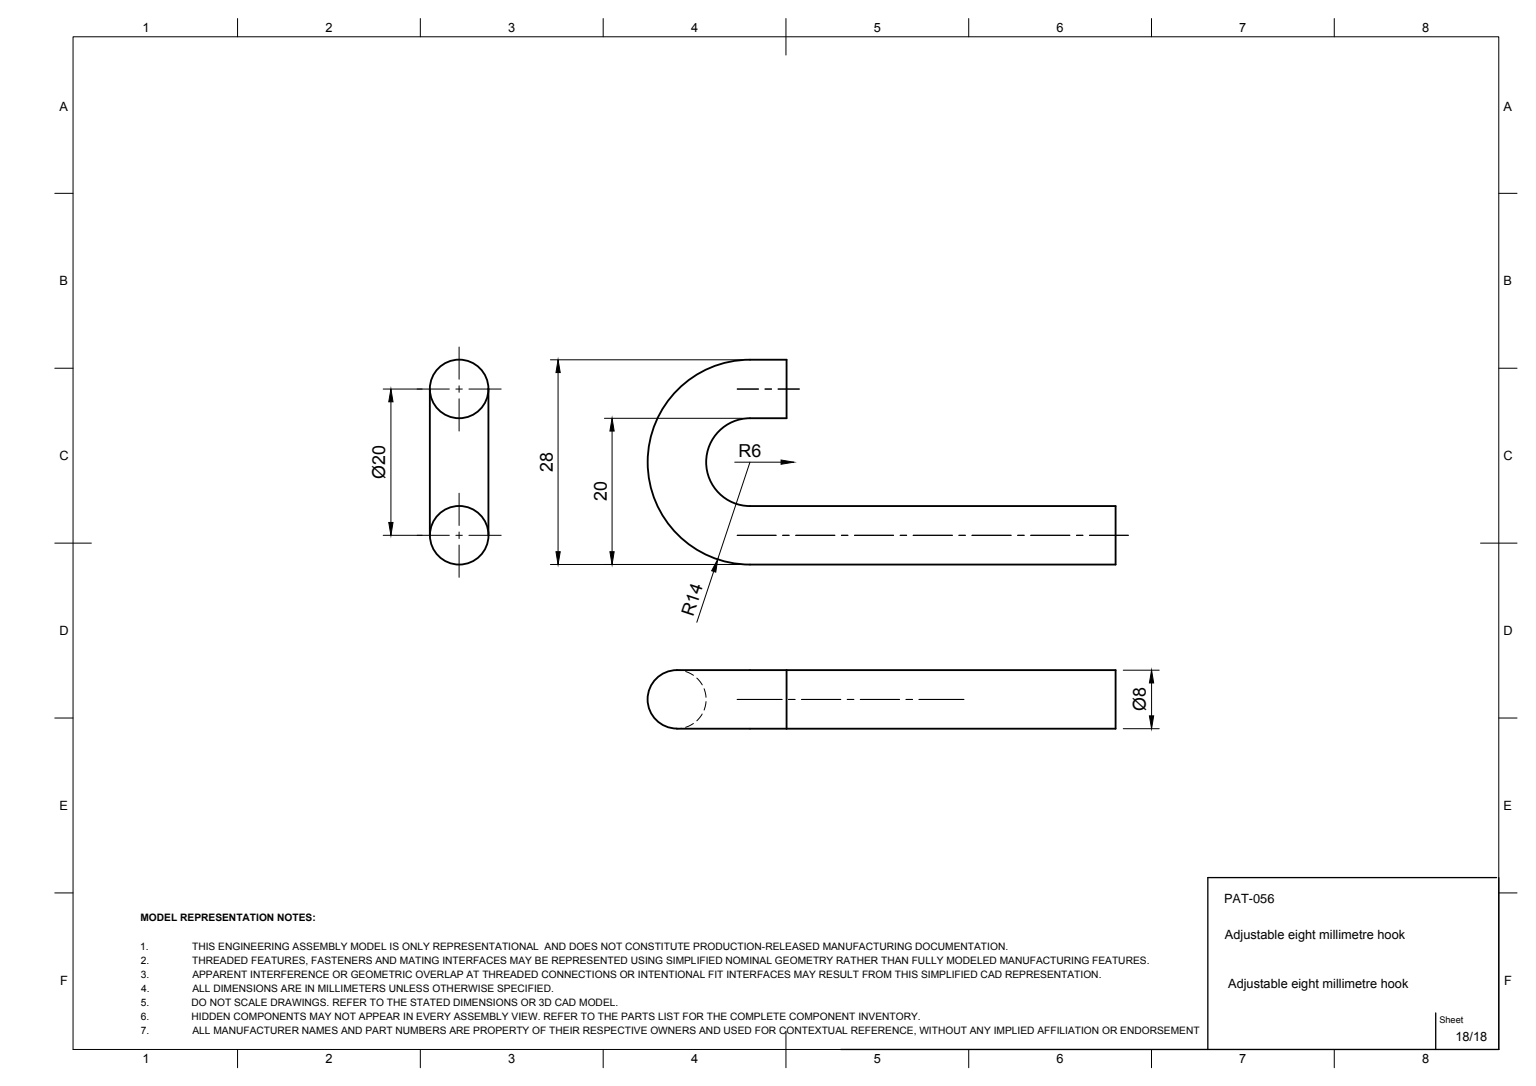
ISO-10303-21;
HEADER;
/* Generated by software containing ST-Developer
 * from STEP Tools, Inc. (www.steptools.com) 
 */

FILE_DESCRIPTION(
/* description */ ('Hook toggle clamp'),
/* implementation_level */ '2;1');

FILE_NAME(
/* name */ 'Adjustable eight millimetre hook.step',
/* time_stamp */ '2026-10-27T21:56:56-07:00',
/* author */ (''),
/* organization */ (''),
/* preprocessor_version */ 'ST-DEVELOPER v20.2',
/* originating_system */ 'Autodesk Translation Framework v15.17.0.0',
/* authorisation */ '');

FILE_SCHEMA (('AUTOMOTIVE_DESIGN { 1 0 10303 214 3 1 1 }'));
ENDSEC;

DATA;
#10=MECHANICAL_DESIGN_GEOMETRIC_PRESENTATION_REPRESENTATION('',(#203),#5458);
#12=TOROIDAL_SURFACE('',#3465,1.,0.4);
#169=SHAPE_REPRESENTATION_RELATIONSHIP('SRR','None',#5553,#186);
#186=ADVANCED_BREP_SHAPE_REPRESENTATION('',(#219),#5455);
#203=STYLED_ITEM('',(#5731),#219);
#219=MANIFOLD_SOLID_BREP('Body1',#2985);
#381=PLANE('',#3471);
#382=PLANE('',#3472);
#546=FACE_OUTER_BOUND('',#771,.T.);
#547=FACE_OUTER_BOUND('',#772,.T.);
#548=FACE_OUTER_BOUND('',#773,.T.);
#549=FACE_OUTER_BOUND('',#774,.T.);
#550=FACE_OUTER_BOUND('',#775,.T.);
#771=EDGE_LOOP('',(#2669,#2670,#2671,#2672,#2673));
#772=EDGE_LOOP('',(#2674,#2675,#2676,#2677,#2678,#2679));
#773=EDGE_LOOP('',(#2680,#2681,#2682,#2683,#2684));
#774=EDGE_LOOP('',(#2685));
#775=EDGE_LOOP('',(#2686));
#1019=LINE('',#5292,#1256);
#1020=LINE('',#5304,#1257);
#1256=VECTOR('',#4309,0.4);
#1257=VECTOR('',#4324,0.4);
#1367=CIRCLE('',#3462,0.4);
#1368=CIRCLE('',#3463,0.4);
#1369=CIRCLE('',#3464,0.4);
#1370=CIRCLE('',#3466,0.6);
#1371=CIRCLE('',#3467,0.4);
#1372=CIRCLE('',#3468,0.4);
#1373=CIRCLE('',#3470,0.4);
#1601=VERTEX_POINT('',#5289);
#1602=VERTEX_POINT('',#5291);
#1603=VERTEX_POINT('',#5293);
#1604=VERTEX_POINT('',#5297);
#1605=VERTEX_POINT('',#5299);
#1606=VERTEX_POINT('',#5303);
#1961=EDGE_CURVE('',#1601,#1601,#1367,.T.);
#1962=EDGE_CURVE('',#1601,#1602,#1019,.T.);
#1963=EDGE_CURVE('',#1602,#1603,#1368,.T.);
#1964=EDGE_CURVE('',#1603,#1602,#1369,.T.);
#1965=EDGE_CURVE('',#1603,#1604,#1370,.T.);
#1966=EDGE_CURVE('',#1604,#1605,#1371,.T.);
#1967=EDGE_CURVE('',#1605,#1604,#1372,.T.);
#1968=EDGE_CURVE('',#1605,#1606,#1020,.T.);
#1969=EDGE_CURVE('',#1606,#1606,#1373,.T.);
#2669=ORIENTED_EDGE('',*,*,#1961,.F.);
#2670=ORIENTED_EDGE('',*,*,#1962,.T.);
#2671=ORIENTED_EDGE('',*,*,#1963,.T.);
#2672=ORIENTED_EDGE('',*,*,#1964,.T.);
#2673=ORIENTED_EDGE('',*,*,#1962,.F.);
#2674=ORIENTED_EDGE('',*,*,#1963,.F.);
#2675=ORIENTED_EDGE('',*,*,#1964,.F.);
#2676=ORIENTED_EDGE('',*,*,#1965,.T.);
#2677=ORIENTED_EDGE('',*,*,#1966,.T.);
#2678=ORIENTED_EDGE('',*,*,#1967,.T.);
#2679=ORIENTED_EDGE('',*,*,#1965,.F.);
#2680=ORIENTED_EDGE('',*,*,#1967,.F.);
#2681=ORIENTED_EDGE('',*,*,#1968,.T.);
#2682=ORIENTED_EDGE('',*,*,#1969,.T.);
#2683=ORIENTED_EDGE('',*,*,#1968,.F.);
#2684=ORIENTED_EDGE('',*,*,#1966,.F.);
#2685=ORIENTED_EDGE('',*,*,#1961,.T.);
#2686=ORIENTED_EDGE('',*,*,#1969,.F.);
#2792=CYLINDRICAL_SURFACE('',#3461,0.4);
#2793=CYLINDRICAL_SURFACE('',#3469,0.4);
#2950=ADVANCED_FACE('',(#546),#2792,.T.);
#2951=ADVANCED_FACE('',(#547),#12,.T.);
#2952=ADVANCED_FACE('',(#548),#2793,.T.);
#2953=ADVANCED_FACE('',(#549),#381,.T.);
#2954=ADVANCED_FACE('',(#550),#382,.F.);
#2985=CLOSED_SHELL('',(#2950,#2951,#2952,#2953,#2954));
#3460=AXIS2_PLACEMENT_3D('',#5287,#4303,#4304);
#3461=AXIS2_PLACEMENT_3D('',#5288,#4305,#4306);
#3462=AXIS2_PLACEMENT_3D('',#5290,#4307,#4308);
#3463=AXIS2_PLACEMENT_3D('',#5294,#4310,#4311);
#3464=AXIS2_PLACEMENT_3D('',#5295,#4312,#4313);
#3465=AXIS2_PLACEMENT_3D('',#5296,#4314,#4315);
#3466=AXIS2_PLACEMENT_3D('',#5298,#4316,#4317);
#3467=AXIS2_PLACEMENT_3D('',#5300,#4318,#4319);
#3468=AXIS2_PLACEMENT_3D('',#5301,#4320,#4321);
#3469=AXIS2_PLACEMENT_3D('',#5302,#4322,#4323);
#3470=AXIS2_PLACEMENT_3D('',#5305,#4325,#4326);
#3471=AXIS2_PLACEMENT_3D('',#5306,#4327,#4328);
#3472=AXIS2_PLACEMENT_3D('',#5307,#4329,#4330);
#4303=DIRECTION('axis',(0.,0.,1.));
#4304=DIRECTION('refdir',(1.,0.,0.));
#4305=DIRECTION('center_axis',(-1.,0.,0.));
#4306=DIRECTION('ref_axis',(0.,1.,0.));
#4307=DIRECTION('center_axis',(-1.,0.,1.22464679914735E-16));
#4308=DIRECTION('ref_axis',(0.,1.,0.));
#4309=DIRECTION('',(1.,0.,0.));
#4310=DIRECTION('center_axis',(-1.,0.,1.22464679914735E-16));
#4311=DIRECTION('ref_axis',(0.,1.,0.));
#4312=DIRECTION('center_axis',(-1.,0.,1.22464679914735E-16));
#4313=DIRECTION('ref_axis',(0.,1.,0.));
#4314=DIRECTION('center_axis',(0.,-1.,0.));
#4315=DIRECTION('ref_axis',(0.,0.,-1.));
#4316=DIRECTION('center_axis',(0.,1.,0.));
#4317=DIRECTION('ref_axis',(0.,0.,-1.));
#4318=DIRECTION('center_axis',(1.,0.,0.));
#4319=DIRECTION('ref_axis',(0.,1.,0.));
#4320=DIRECTION('center_axis',(1.,0.,0.));
#4321=DIRECTION('ref_axis',(0.,1.,0.));
#4322=DIRECTION('center_axis',(1.,0.,0.));
#4323=DIRECTION('ref_axis',(0.,1.,0.));
#4324=DIRECTION('',(-1.,0.,0.));
#4325=DIRECTION('center_axis',(1.,0.,0.));
#4326=DIRECTION('ref_axis',(0.,1.,0.));
#4327=DIRECTION('center_axis',(-1.,0.,1.22464679914735E-16));
#4328=DIRECTION('ref_axis',(0.,1.,0.));
#4329=DIRECTION('center_axis',(1.,0.,0.));
#4330=DIRECTION('ref_axis',(0.,1.,0.));
#5287=CARTESIAN_POINT('',(0.,0.,0.));
#5288=CARTESIAN_POINT('Origin',(15.,0.,4.5));
#5289=CARTESIAN_POINT('',(14.5,-0.4,4.5));
#5290=CARTESIAN_POINT('Origin',(14.5,0.,4.5));
#5291=CARTESIAN_POINT('',(15.,-0.4,4.5));
#5292=CARTESIAN_POINT('',(15.,-0.4,4.5));
#5293=CARTESIAN_POINT('',(15.,4.89858719658941E-17,4.1));
#5294=CARTESIAN_POINT('Origin',(15.,0.,4.5));
#5295=CARTESIAN_POINT('Origin',(15.,0.,4.5));
#5296=CARTESIAN_POINT('Origin',(15.,0.,3.5));
#5297=CARTESIAN_POINT('',(15.,4.89858719658941E-17,2.9));
#5298=CARTESIAN_POINT('Origin',(15.,4.89858719658941E-17,3.5));
#5299=CARTESIAN_POINT('',(15.,-0.4,2.5));
#5300=CARTESIAN_POINT('Origin',(15.,0.,2.5));
#5301=CARTESIAN_POINT('Origin',(15.,0.,2.5));
#5302=CARTESIAN_POINT('Origin',(10.,0.,2.5));
#5303=CARTESIAN_POINT('',(10.,-0.4,2.5));
#5304=CARTESIAN_POINT('',(10.,-0.4,2.5));
#5305=CARTESIAN_POINT('Origin',(10.,0.,2.5));
#5306=CARTESIAN_POINT('Origin',(14.5,0.,4.5));
#5307=CARTESIAN_POINT('Origin',(10.,0.,2.5));
#5432=UNCERTAINTY_MEASURE_WITH_UNIT(LENGTH_MEASURE(0.001),#5459,
'DISTANCE_ACCURACY_VALUE',
'Maximum model space distance between geometric entities at asserted c
onnectivities');
#5435=UNCERTAINTY_MEASURE_WITH_UNIT(LENGTH_MEASURE(0.001),#5459,
'DISTANCE_ACCURACY_VALUE',
'Maximum model space distance between geometric entities at asserted c
onnectivities');
#5455=(
GEOMETRIC_REPRESENTATION_CONTEXT(3)
GLOBAL_UNCERTAINTY_ASSIGNED_CONTEXT((#5432))
GLOBAL_UNIT_ASSIGNED_CONTEXT((#5459,#5461,#5462))
REPRESENTATION_CONTEXT('','3D')
);
#5458=(
GEOMETRIC_REPRESENTATION_CONTEXT(3)
GLOBAL_UNCERTAINTY_ASSIGNED_CONTEXT((#5435))
GLOBAL_UNIT_ASSIGNED_CONTEXT((#5459,#5461,#5462))
REPRESENTATION_CONTEXT('','3D')
);
#5459=(
LENGTH_UNIT()
NAMED_UNIT(*)
SI_UNIT(.CENTI.,.METRE.)
);
#5461=(
NAMED_UNIT(*)
PLANE_ANGLE_UNIT()
SI_UNIT($,.RADIAN.)
);
#5462=(
NAMED_UNIT(*)
SI_UNIT($,.STERADIAN.)
SOLID_ANGLE_UNIT()
);
#5482=SHAPE_DEFINITION_REPRESENTATION(#5518,#5553);
#5518=PRODUCT_DEFINITION_SHAPE('',$,#5576);
#5553=SHAPE_REPRESENTATION('',(#3460),#5455);
#5556=PRODUCT_DEFINITION_CONTEXT('part definition',#5624,'design');
#5576=PRODUCT_DEFINITION('Adjustable eight millimetre hook',
'Adjustable eight millimetre hook',#5598,#5556);
#5598=PRODUCT_DEFINITION_FORMATION('',$,#5645);
#5624=APPLICATION_CONTEXT(
'Core Data for Automotive Mechanical Design Process');
#5625=PRODUCT_CONTEXT('part definition',#5624,'mechanical');
#5645=PRODUCT('Adjustable eight millimetre hook',
'Adjustable eight millimetre hook','Adjustable eight millimetre hook',(#5625));
#5725=COLOUR_RGB('Off White',0.89,0.88,0.83);
#5726=FILL_AREA_STYLE_COLOUR('',#5725);
#5727=FILL_AREA_STYLE('',(#5726));
#5728=SURFACE_STYLE_FILL_AREA(#5727);
#5729=SURFACE_SIDE_STYLE('',(#5728));
#5730=SURFACE_STYLE_USAGE(.BOTH.,#5729);
#5731=PRESENTATION_STYLE_ASSIGNMENT((#5730));
ENDSEC;
END-ISO-10303-21;
